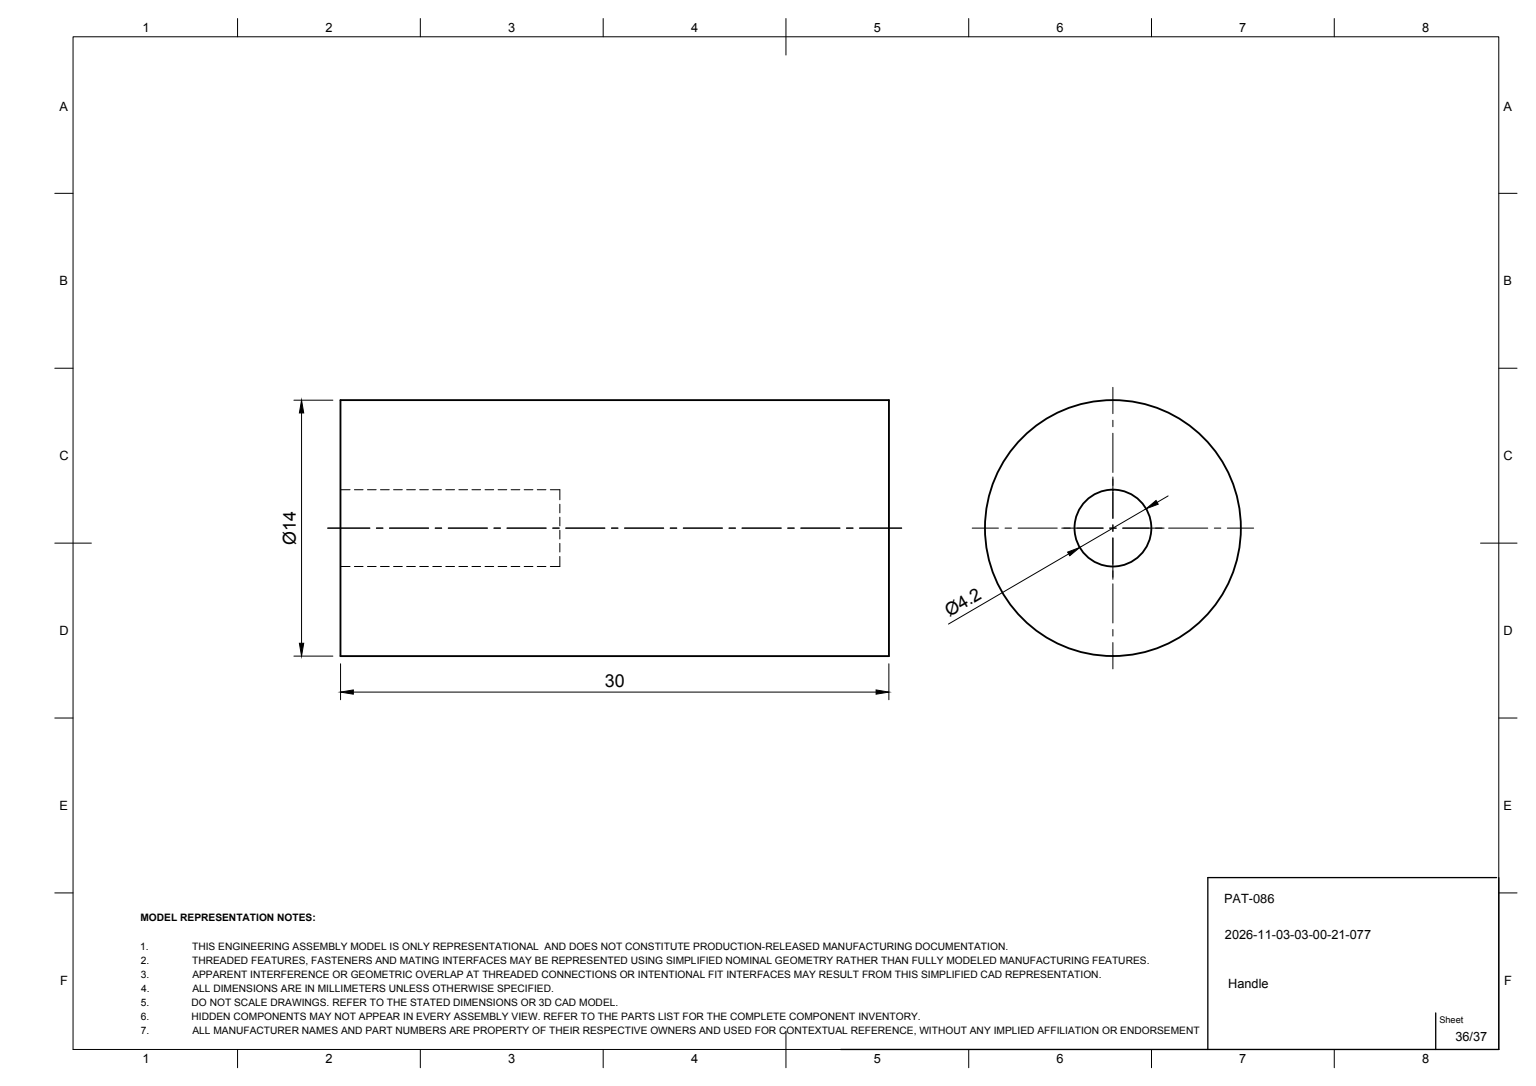
ISO-10303-21;
HEADER;
/* Generated by software containing ST-Developer
 * from STEP Tools, Inc. (www.steptools.com) 
 */

FILE_DESCRIPTION(
/* description */ ('Ratchet and pawl hand winch drum'),
/* implementation_level */ '2;1');

FILE_NAME(
/* name */ 'Handle.step',
/* time_stamp */ '2026-10-27T12:42:58-07:00',
/* author */ (''),
/* organization */ (''),
/* preprocessor_version */ 'ST-DEVELOPER v20.2',
/* originating_system */ 'Autodesk Translation Framework v15.17.0.0',
/* authorisation */ '');

FILE_SCHEMA (('AUTOMOTIVE_DESIGN { 1 0 10303 214 3 1 1 }'));
ENDSEC;

DATA;
#10=MECHANICAL_DESIGN_GEOMETRIC_PRESENTATION_REPRESENTATION('',(#420),#11801);
#351=SHAPE_REPRESENTATION_RELATIONSHIP('SRR','None',#11979,#385);
#385=ADVANCED_BREP_SHAPE_REPRESENTATION('',(#453),#11796);
#420=STYLED_ITEM('',(#12206),#453);
#453=MANIFOLD_SOLID_BREP('Body1',#6299);
#596=FACE_BOUND('',#1655,.T.);
#812=PLANE('',#7237);
#813=PLANE('',#7241);
#814=PLANE('',#7242);
#1155=FACE_OUTER_BOUND('',#1651,.T.);
#1156=FACE_OUTER_BOUND('',#1652,.T.);
#1157=FACE_OUTER_BOUND('',#1653,.T.);
#1158=FACE_OUTER_BOUND('',#1654,.T.);
#1159=FACE_OUTER_BOUND('',#1656,.T.);
#1651=EDGE_LOOP('',(#5651,#5652,#5653,#5654));
#1652=EDGE_LOOP('',(#5655));
#1653=EDGE_LOOP('',(#5656,#5657,#5658,#5659));
#1654=EDGE_LOOP('',(#5660));
#1655=EDGE_LOOP('',(#5661));
#1656=EDGE_LOOP('',(#5662));
#2150=LINE('',#11494,#2661);
#2151=LINE('',#11501,#2662);
#2661=VECTOR('',#8925,0.21);
#2662=VECTOR('',#8934,0.7);
#2922=CIRCLE('',#7235,0.21);
#2923=CIRCLE('',#7236,0.21);
#2924=CIRCLE('',#7239,0.7);
#2925=CIRCLE('',#7240,0.7);
#3417=VERTEX_POINT('',#11491);
#3418=VERTEX_POINT('',#11493);
#3419=VERTEX_POINT('',#11498);
#3420=VERTEX_POINT('',#11500);
#4169=EDGE_CURVE('',#3417,#3417,#2922,.T.);
#4170=EDGE_CURVE('',#3417,#3418,#2150,.T.);
#4171=EDGE_CURVE('',#3418,#3418,#2923,.T.);
#4172=EDGE_CURVE('',#3419,#3419,#2924,.T.);
#4173=EDGE_CURVE('',#3419,#3420,#2151,.T.);
#4174=EDGE_CURVE('',#3420,#3420,#2925,.T.);
#5651=ORIENTED_EDGE('',*,*,#4169,.F.);
#5652=ORIENTED_EDGE('',*,*,#4170,.T.);
#5653=ORIENTED_EDGE('',*,*,#4171,.F.);
#5654=ORIENTED_EDGE('',*,*,#4170,.F.);
#5655=ORIENTED_EDGE('',*,*,#4169,.T.);
#5656=ORIENTED_EDGE('',*,*,#4172,.F.);
#5657=ORIENTED_EDGE('',*,*,#4173,.T.);
#5658=ORIENTED_EDGE('',*,*,#4174,.T.);
#5659=ORIENTED_EDGE('',*,*,#4173,.F.);
#5660=ORIENTED_EDGE('',*,*,#4172,.T.);
#5661=ORIENTED_EDGE('',*,*,#4171,.T.);
#5662=ORIENTED_EDGE('',*,*,#4174,.F.);
#5903=CYLINDRICAL_SURFACE('',#7234,0.21);
#5904=CYLINDRICAL_SURFACE('',#7238,0.7);
#6225=ADVANCED_FACE('',(#1155),#5903,.F.);
#6226=ADVANCED_FACE('',(#1156),#812,.T.);
#6227=ADVANCED_FACE('',(#1157),#5904,.T.);
#6228=ADVANCED_FACE('',(#1158,#596),#813,.T.);
#6229=ADVANCED_FACE('',(#1159),#814,.F.);
#6299=CLOSED_SHELL('',(#6225,#6226,#6227,#6228,#6229));
#7233=AXIS2_PLACEMENT_3D('',#11489,#8919,#8920);
#7234=AXIS2_PLACEMENT_3D('',#11490,#8921,#8922);
#7235=AXIS2_PLACEMENT_3D('',#11492,#8923,#8924);
#7236=AXIS2_PLACEMENT_3D('',#11495,#8926,#8927);
#7237=AXIS2_PLACEMENT_3D('',#11496,#8928,#8929);
#7238=AXIS2_PLACEMENT_3D('',#11497,#8930,#8931);
#7239=AXIS2_PLACEMENT_3D('',#11499,#8932,#8933);
#7240=AXIS2_PLACEMENT_3D('',#11502,#8935,#8936);
#7241=AXIS2_PLACEMENT_3D('',#11503,#8937,#8938);
#7242=AXIS2_PLACEMENT_3D('',#11504,#8939,#8940);
#8919=DIRECTION('axis',(0.,0.,1.));
#8920=DIRECTION('refdir',(1.,0.,0.));
#8921=DIRECTION('center_axis',(0.,1.,0.));
#8922=DIRECTION('ref_axis',(1.,0.,0.));
#8923=DIRECTION('center_axis',(0.,1.,0.));
#8924=DIRECTION('ref_axis',(1.,0.,0.));
#8925=DIRECTION('',(0.,1.,0.));
#8926=DIRECTION('center_axis',(0.,-1.,0.));
#8927=DIRECTION('ref_axis',(1.,0.,0.));
#8928=DIRECTION('center_axis',(0.,1.,0.));
#8929=DIRECTION('ref_axis',(1.,0.,0.));
#8930=DIRECTION('center_axis',(0.,1.,0.));
#8931=DIRECTION('ref_axis',(1.,0.,0.));
#8932=DIRECTION('center_axis',(0.,1.,0.));
#8933=DIRECTION('ref_axis',(1.,0.,0.));
#8934=DIRECTION('',(0.,-1.,0.));
#8935=DIRECTION('center_axis',(0.,1.,0.));
#8936=DIRECTION('ref_axis',(1.,0.,0.));
#8937=DIRECTION('center_axis',(0.,1.,0.));
#8938=DIRECTION('ref_axis',(1.,0.,0.));
#8939=DIRECTION('center_axis',(0.,1.,0.));
#8940=DIRECTION('ref_axis',(1.,0.,0.));
#11489=CARTESIAN_POINT('',(0.,0.,0.));
#11490=CARTESIAN_POINT('Origin',(0.,-7.7,10.03));
#11491=CARTESIAN_POINT('',(-0.21,-7.7,10.03));
#11492=CARTESIAN_POINT('Origin',(0.,-7.7,10.03));
#11493=CARTESIAN_POINT('',(-0.21,-6.5,10.03));
#11494=CARTESIAN_POINT('',(-0.21,-7.7,10.03));
#11495=CARTESIAN_POINT('Origin',(0.,-6.5,10.03));
#11496=CARTESIAN_POINT('Origin',(0.,-7.7,10.03));
#11497=CARTESIAN_POINT('Origin',(0.,-9.5,10.03));
#11498=CARTESIAN_POINT('',(-0.7,-6.5,10.03));
#11499=CARTESIAN_POINT('Origin',(0.,-6.5,10.03));
#11500=CARTESIAN_POINT('',(-0.7,-9.5,10.03));
#11501=CARTESIAN_POINT('',(-0.7,-9.5,10.03));
#11502=CARTESIAN_POINT('Origin',(0.,-9.5,10.03));
#11503=CARTESIAN_POINT('Origin',(0.,-6.5,10.03));
#11504=CARTESIAN_POINT('Origin',(0.,-9.5,10.03));
#11756=UNCERTAINTY_MEASURE_WITH_UNIT(LENGTH_MEASURE(0.001),#11802,
'DISTANCE_ACCURACY_VALUE',
'Maximum model space distance between geometric entities at asserted c
onnectivities');
#11761=UNCERTAINTY_MEASURE_WITH_UNIT(LENGTH_MEASURE(0.001),#11802,
'DISTANCE_ACCURACY_VALUE',
'Maximum model space distance between geometric entities at asserted c
onnectivities');
#11796=(
GEOMETRIC_REPRESENTATION_CONTEXT(3)
GLOBAL_UNCERTAINTY_ASSIGNED_CONTEXT((#11756))
GLOBAL_UNIT_ASSIGNED_CONTEXT((#11802,#11804,#11805))
REPRESENTATION_CONTEXT('','3D')
);
#11801=(
GEOMETRIC_REPRESENTATION_CONTEXT(3)
GLOBAL_UNCERTAINTY_ASSIGNED_CONTEXT((#11761))
GLOBAL_UNIT_ASSIGNED_CONTEXT((#11802,#11804,#11805))
REPRESENTATION_CONTEXT('','3D')
);
#11802=(
LENGTH_UNIT()
NAMED_UNIT(*)
SI_UNIT(.CENTI.,.METRE.)
);
#11804=(
NAMED_UNIT(*)
PLANE_ANGLE_UNIT()
SI_UNIT($,.RADIAN.)
);
#11805=(
NAMED_UNIT(*)
SI_UNIT($,.STERADIAN.)
SOLID_ANGLE_UNIT()
);
#11840=SHAPE_DEFINITION_REPRESENTATION(#11881,#11979);
#11881=PRODUCT_DEFINITION_SHAPE('',$,#12019);
#11979=SHAPE_REPRESENTATION('',(#7233),#11796);
#11984=PRODUCT_DEFINITION_CONTEXT('part definition',#12103,'design');
#12019=PRODUCT_DEFINITION('Handle','Handle',#12058,#11984);
#12058=PRODUCT_DEFINITION_FORMATION('',$,#12139);
#12103=APPLICATION_CONTEXT(
'Core Data for Automotive Mechanical Design Process');
#12104=PRODUCT_CONTEXT('part definition',#12103,'mechanical');
#12139=PRODUCT('Handle','Handle','Handle',(#12104));
#12200=COLOUR_RGB('Sky Blue',0.24,0.69,0.87);
#12201=FILL_AREA_STYLE_COLOUR('',#12200);
#12202=FILL_AREA_STYLE('',(#12201));
#12203=SURFACE_STYLE_FILL_AREA(#12202);
#12204=SURFACE_SIDE_STYLE('',(#12203));
#12205=SURFACE_STYLE_USAGE(.BOTH.,#12204);
#12206=PRESENTATION_STYLE_ASSIGNMENT((#12205));
ENDSEC;
END-ISO-10303-21;
